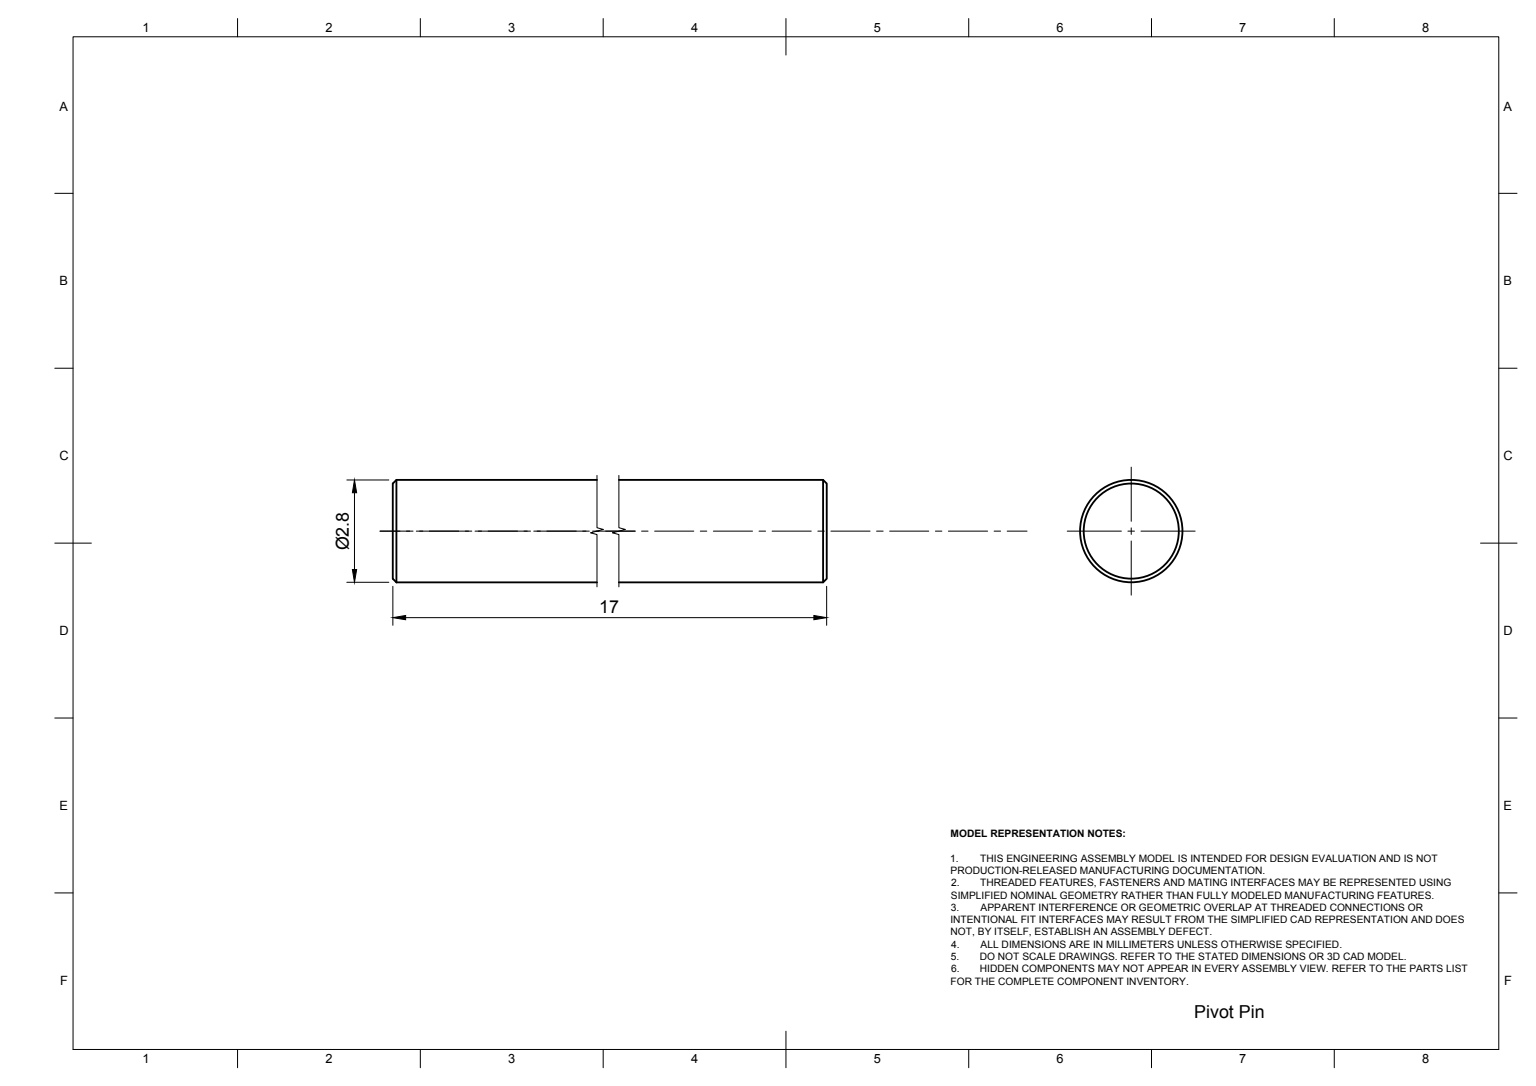
ISO-10303-21;
HEADER;
/* Generated by software containing ST-Developer
 * from STEP Tools, Inc. (www.steptools.com) 
 */

FILE_DESCRIPTION(
/* description */ ('STEP AP214'),
/* implementation_level */ '2;1');

FILE_NAME(
/* name */ 'Pivot Pin.step',
/* time_stamp */ '2026-10-06T00:19:40-07:00',
/* author */ (''),
/* organization */ (''),
/* preprocessor_version */ 'ST-DEVELOPER v20.2',
/* originating_system */ 'Autodesk Translation Framework v15.15.0.0',
/* authorisation */ '');

FILE_SCHEMA (('AUTOMOTIVE_DESIGN { 1 0 10303 214 3 1 1 }'));
ENDSEC;

DATA;
#10=MECHANICAL_DESIGN_GEOMETRIC_PRESENTATION_REPRESENTATION('',(#2063),#98302);
#2043=SHAPE_REPRESENTATION_RELATIONSHIP('SRR','None',#98340,#2053);
#2053=ADVANCED_BREP_SHAPE_REPRESENTATION('',(#2073),#98292);
#2063=STYLED_ITEM('',(#98399),#2073);
#2073=MANIFOLD_SOLID_BREP('Body1',#34167);
#2082=PLANE('',#34299);
#2083=PLANE('',#34302);
#2521=CYLINDRICAL_SURFACE('',#34296,1.4);
#3279=FACE_OUTER_BOUND('',#5419,.T.);
#3280=FACE_OUTER_BOUND('',#5420,.T.);
#3281=FACE_OUTER_BOUND('',#5421,.T.);
#3282=FACE_OUTER_BOUND('',#5422,.T.);
#3283=FACE_OUTER_BOUND('',#5423,.T.);
#5419=EDGE_LOOP('',(#21783,#21784,#21785,#21786,#21787));
#5420=EDGE_LOOP('',(#21788,#21789,#21790,#21791,#21792,#21793));
#5421=EDGE_LOOP('',(#21794));
#5422=EDGE_LOOP('',(#21795,#21796,#21797,#21798,#21799));
#5423=EDGE_LOOP('',(#21800));
#7637=LINE('',#49115,#9477);
#7638=LINE('',#49122,#9478);
#7639=LINE('',#49127,#9479);
#9477=VECTOR('',#38624,0.999999999999103);
#9478=VECTOR('',#38633,1.4);
#9479=VECTOR('',#38640,0.999999999999103);
#11317=CIRCLE('',#34293,1.4);
#11318=CIRCLE('',#34294,1.3);
#11319=CIRCLE('',#34295,1.4);
#11320=CIRCLE('',#34297,1.4);
#11321=CIRCLE('',#34298,1.4);
#11322=CIRCLE('',#34301,1.3);
#13625=VERTEX_POINT('',#49111);
#13626=VERTEX_POINT('',#49112);
#13627=VERTEX_POINT('',#49114);
#13628=VERTEX_POINT('',#49119);
#13629=VERTEX_POINT('',#49120);
#13630=VERTEX_POINT('',#49126);
#16663=EDGE_CURVE('',#13625,#13626,#11317,.T.);
#16664=EDGE_CURVE('',#13625,#13627,#7637,.T.);
#16665=EDGE_CURVE('',#13627,#13627,#11318,.T.);
#16666=EDGE_CURVE('',#13626,#13625,#11319,.T.);
#16667=EDGE_CURVE('',#13628,#13629,#11320,.T.);
#16668=EDGE_CURVE('',#13628,#13626,#7638,.T.);
#16669=EDGE_CURVE('',#13629,#13628,#11321,.T.);
#16670=EDGE_CURVE('',#13629,#13630,#7639,.T.);
#16671=EDGE_CURVE('',#13630,#13630,#11322,.T.);
#21783=ORIENTED_EDGE('',*,*,#16663,.F.);
#21784=ORIENTED_EDGE('',*,*,#16664,.T.);
#21785=ORIENTED_EDGE('',*,*,#16665,.T.);
#21786=ORIENTED_EDGE('',*,*,#16664,.F.);
#21787=ORIENTED_EDGE('',*,*,#16666,.F.);
#21788=ORIENTED_EDGE('',*,*,#16667,.F.);
#21789=ORIENTED_EDGE('',*,*,#16668,.T.);
#21790=ORIENTED_EDGE('',*,*,#16666,.T.);
#21791=ORIENTED_EDGE('',*,*,#16663,.T.);
#21792=ORIENTED_EDGE('',*,*,#16668,.F.);
#21793=ORIENTED_EDGE('',*,*,#16669,.F.);
#21794=ORIENTED_EDGE('',*,*,#16665,.F.);
#21795=ORIENTED_EDGE('',*,*,#16667,.T.);
#21796=ORIENTED_EDGE('',*,*,#16670,.T.);
#21797=ORIENTED_EDGE('',*,*,#16671,.F.);
#21798=ORIENTED_EDGE('',*,*,#16670,.F.);
#21799=ORIENTED_EDGE('',*,*,#16669,.T.);
#21800=ORIENTED_EDGE('',*,*,#16671,.T.);
#32023=CONICAL_SURFACE('',#34292,0.999999999999103,0.785398163397);
#32024=CONICAL_SURFACE('',#34300,0.999999999999103,0.785398163397);
#32027=ADVANCED_FACE('',(#3279),#32023,.T.);
#32028=ADVANCED_FACE('',(#3280),#2521,.T.);
#32029=ADVANCED_FACE('',(#3281),#2082,.F.);
#32030=ADVANCED_FACE('',(#3282),#32024,.T.);
#32031=ADVANCED_FACE('',(#3283),#2083,.T.);
#34167=CLOSED_SHELL('',(#32027,#32028,#32029,#32030,#32031));
#34291=AXIS2_PLACEMENT_3D('',#49109,#38618,#38619);
#34292=AXIS2_PLACEMENT_3D('',#49110,#38620,#38621);
#34293=AXIS2_PLACEMENT_3D('',#49113,#38622,#38623);
#34294=AXIS2_PLACEMENT_3D('',#49116,#38625,#38626);
#34295=AXIS2_PLACEMENT_3D('',#49117,#38627,#38628);
#34296=AXIS2_PLACEMENT_3D('',#49118,#38629,#38630);
#34297=AXIS2_PLACEMENT_3D('',#49121,#38631,#38632);
#34298=AXIS2_PLACEMENT_3D('',#49123,#38634,#38635);
#34299=AXIS2_PLACEMENT_3D('',#49124,#38636,#38637);
#34300=AXIS2_PLACEMENT_3D('',#49125,#38638,#38639);
#34301=AXIS2_PLACEMENT_3D('',#49128,#38641,#38642);
#34302=AXIS2_PLACEMENT_3D('',#49129,#38643,#38644);
#38618=DIRECTION('axis',(0.,0.,1.));
#38619=DIRECTION('refdir',(1.,0.,0.));
#38620=DIRECTION('center_axis',(1.,-1.7744788353171E-14,4.9634756259259E-15));
#38621=DIRECTION('ref_axis',(-1.3170890159705E-14,-0.50000000000019,0.866025403784329));
#38622=DIRECTION('center_axis',(1.,0.,0.));
#38623=DIRECTION('ref_axis',(0.,1.,0.));
#38624=DIRECTION('',(-0.707106781186874,-0.353553390593237,0.612372435695439));
#38625=DIRECTION('center_axis',(1.,0.,0.));
#38626=DIRECTION('ref_axis',(0.,1.,0.));
#38627=DIRECTION('center_axis',(1.,0.,0.));
#38628=DIRECTION('ref_axis',(0.,1.,0.));
#38629=DIRECTION('center_axis',(1.,0.,0.));
#38630=DIRECTION('ref_axis',(0.,1.,0.));
#38631=DIRECTION('center_axis',(1.,1.11593432733E-14,6.44284984283E-15));
#38632=DIRECTION('ref_axis',(-1.11593432733E-14,1.,-4.86402894982592E-32));
#38633=DIRECTION('',(-1.,0.,0.));
#38634=DIRECTION('center_axis',(1.,1.11593432733E-14,6.44284984283E-15));
#38635=DIRECTION('ref_axis',(-1.11593432733E-14,1.,-4.86402894982592E-32));
#38636=DIRECTION('center_axis',(1.,0.,0.));
#38637=DIRECTION('ref_axis',(0.,1.,0.));
#38638=DIRECTION('center_axis',(-1.,-1.7744788353171E-14,4.9634756259259E-15));
#38639=DIRECTION('ref_axis',(1.3170890159705E-14,-0.50000000000019,0.866025403784329));
#38640=DIRECTION('',(0.707106781186874,-0.353553390593237,0.612372435695439));
#38641=DIRECTION('center_axis',(1.,0.,0.));
#38642=DIRECTION('ref_axis',(0.,1.,0.));
#38643=DIRECTION('center_axis',(1.,0.,0.));
#38644=DIRECTION('ref_axis',(0.,1.,0.));
#49109=CARTESIAN_POINT('',(0.,0.,0.));
#49110=CARTESIAN_POINT('Origin',(-8.8,-9.17423561284002,0.473661560390005));
#49111=CARTESIAN_POINT('',(-8.39999999999935,-8.47423561284007,-0.738774004907511));
#49112=CARTESIAN_POINT('',(-8.4,-10.57423561284,0.47366156039));
#49113=CARTESIAN_POINT('Origin',(-8.4,-9.17423561284,0.47366156039));
#49114=CARTESIAN_POINT('',(-8.4999999999994,-8.52423561284007,-0.652171464529114));
#49115=CARTESIAN_POINT('',(-8.79999999999999,-8.67423561284028,-0.392363843393547));
#49116=CARTESIAN_POINT('Origin',(-8.5,-9.17423561284,0.47366156039));
#49117=CARTESIAN_POINT('Origin',(-8.4,-9.17423561284,0.47366156039));
#49118=CARTESIAN_POINT('Origin',(0.,-9.17423561284,0.47366156039));
#49119=CARTESIAN_POINT('',(8.4,-10.5742356128,0.47366156039));
#49120=CARTESIAN_POINT('',(8.39999999999934,-8.47423561284007,-0.73877400490752));
#49121=CARTESIAN_POINT('Origin',(8.4,-9.17423561284,0.47366156039));
#49122=CARTESIAN_POINT('',(0.,-10.57423561284,0.47366156039));
#49123=CARTESIAN_POINT('Origin',(8.4,-9.17423561284,0.47366156039));
#49124=CARTESIAN_POINT('Origin',(-8.5,0.,0.));
#49125=CARTESIAN_POINT('Origin',(8.8,-9.17423561284002,0.473661560390005));
#49126=CARTESIAN_POINT('',(8.4999999999994,-8.52423561284007,-0.652171464529115));
#49127=CARTESIAN_POINT('',(8.79999999999999,-8.67423561284028,-0.392363843393547));
#49128=CARTESIAN_POINT('Origin',(8.5,-9.17423561284,0.47366156039));
#49129=CARTESIAN_POINT('Origin',(8.5,0.,0.));
#98280=UNCERTAINTY_MEASURE_WITH_UNIT(LENGTH_MEASURE(0.01),#98303,
'DISTANCE_ACCURACY_VALUE',
'Maximum model space distance between geometric entities at asserted c
onnectivities');
#98290=UNCERTAINTY_MEASURE_WITH_UNIT(LENGTH_MEASURE(0.01),#98303,
'DISTANCE_ACCURACY_VALUE',
'Maximum model space distance between geometric entities at asserted c
onnectivities');
#98292=(
GEOMETRIC_REPRESENTATION_CONTEXT(3)
GLOBAL_UNCERTAINTY_ASSIGNED_CONTEXT((#98280))
GLOBAL_UNIT_ASSIGNED_CONTEXT((#98303,#98305,#98306))
REPRESENTATION_CONTEXT('','3D')
);
#98302=(
GEOMETRIC_REPRESENTATION_CONTEXT(3)
GLOBAL_UNCERTAINTY_ASSIGNED_CONTEXT((#98290))
GLOBAL_UNIT_ASSIGNED_CONTEXT((#98303,#98305,#98306))
REPRESENTATION_CONTEXT('','3D')
);
#98303=(
LENGTH_UNIT()
NAMED_UNIT(*)
SI_UNIT(.MILLI.,.METRE.)
);
#98305=(
NAMED_UNIT(*)
PLANE_ANGLE_UNIT()
SI_UNIT($,.RADIAN.)
);
#98306=(
NAMED_UNIT(*)
SI_UNIT($,.STERADIAN.)
SOLID_ANGLE_UNIT()
);
#98308=SHAPE_DEFINITION_REPRESENTATION(#98319,#98340);
#98319=PRODUCT_DEFINITION_SHAPE('',$,#98352);
#98340=SHAPE_REPRESENTATION('',(#34291),#98292);
#98350=PRODUCT_DEFINITION_CONTEXT('part definition',#98385,'design');
#98352=PRODUCT_DEFINITION('Pivot Pin','Pivot Pin',#98363,#98350);
#98363=PRODUCT_DEFINITION_FORMATION('',$,#98388);
#98385=APPLICATION_CONTEXT(
'Core Data for Automotive Mechanical Design Process');
#98386=PRODUCT_CONTEXT('part definition',#98385,'mechanical');
#98388=PRODUCT('Pivot Pin','Pivot Pin',$,(#98386));
#98399=PRESENTATION_STYLE_ASSIGNMENT((#98401));
#98401=SURFACE_STYLE_USAGE(.BOTH.,#98403);
#98403=SURFACE_SIDE_STYLE('',(#98405));
#98405=SURFACE_STYLE_FILL_AREA(#98407);
#98407=FILL_AREA_STYLE('Opaque(202,209,238)',(#98409));
#98409=FILL_AREA_STYLE_COLOUR('Opaque(202,209,238)',#98411);
#98411=COLOUR_RGB('Opaque(202,209,238)', 0.31764706, 0.68627451, 0.89019608);
ENDSEC;
END-ISO-10303-21;
